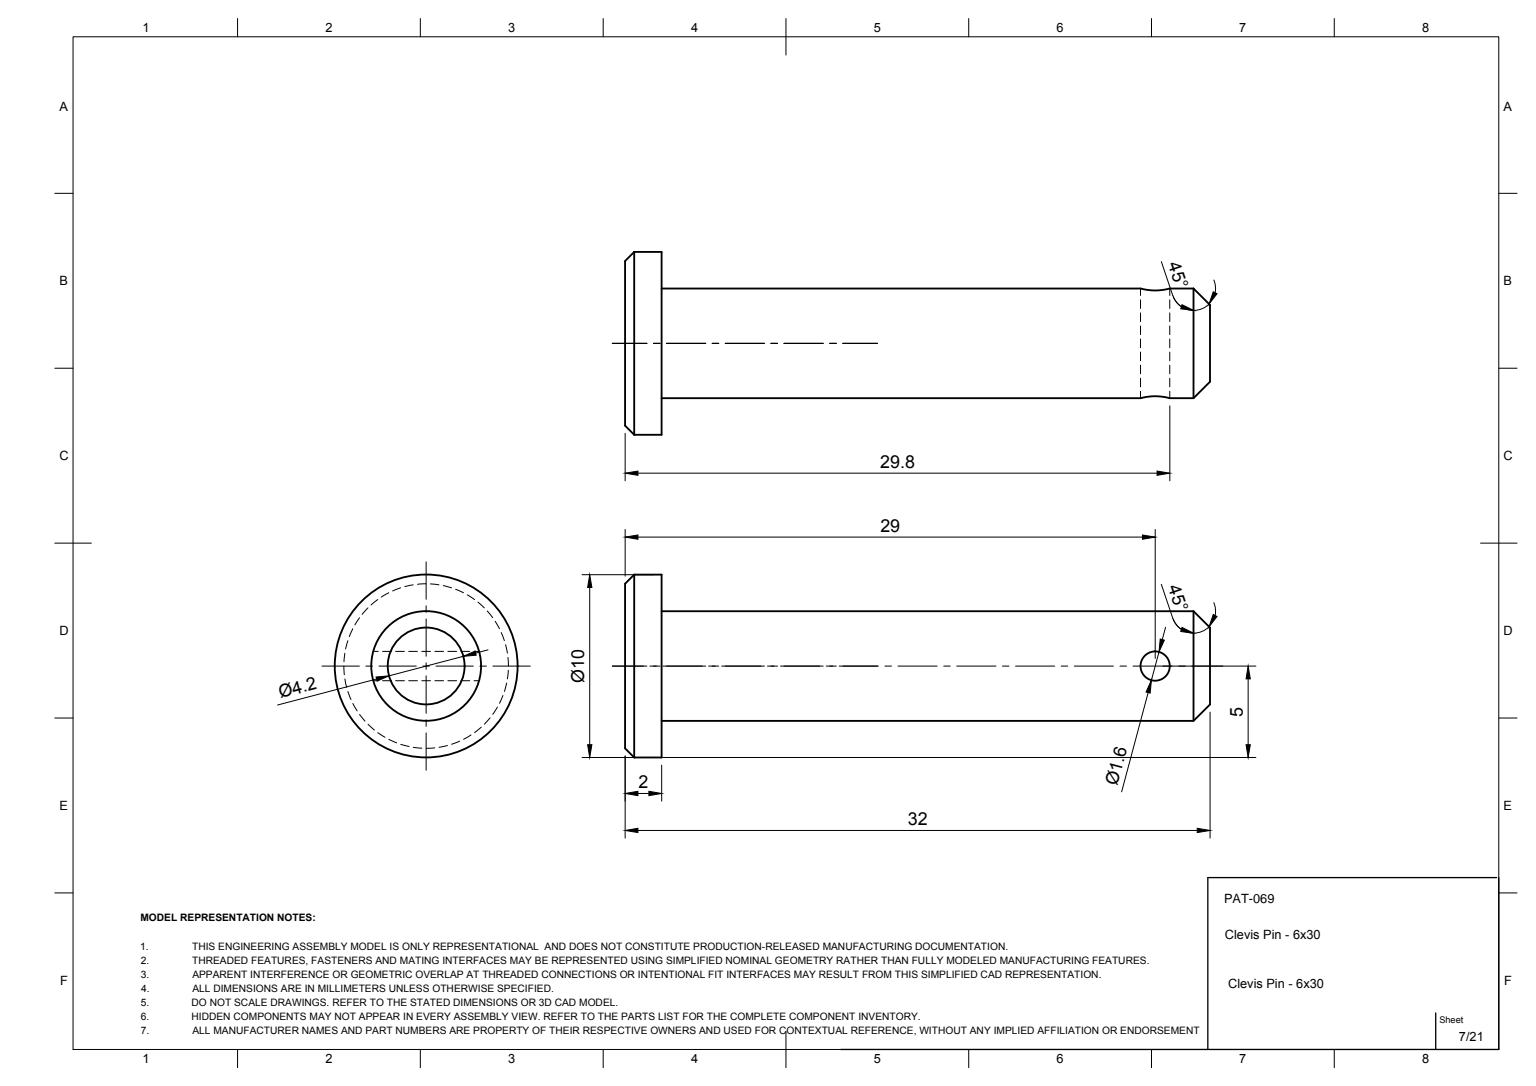
ISO-10303-21;
HEADER;
/* Generated by software containing ST-Developer
 * from STEP Tools, Inc. (www.steptools.com) 
 */

FILE_DESCRIPTION(
/* description */ ('Located fixture plate with toggle clamp'),
/* implementation_level */ '2;1');

FILE_NAME(
/* name */ 'Clevis Pin - 6x30.step',
/* time_stamp */ '2026-10-27T21:36:12-07:00',
/* author */ (''),
/* organization */ (''),
/* preprocessor_version */ 'ST-DEVELOPER v20.2',
/* originating_system */ 'Autodesk Translation Framework v15.17.0.0',
/* authorisation */ '');

FILE_SCHEMA (('AUTOMOTIVE_DESIGN { 1 0 10303 214 3 1 1 }'));
ENDSEC;

DATA;
#10=MECHANICAL_DESIGN_GEOMETRIC_PRESENTATION_REPRESENTATION('',(#341),#9285);
#12=B_SPLINE_CURVE_WITH_KNOTS('',3,(#8976,#8977,#8978,#8979,#8980,#8981,
#8982,#8983,#8984,#8985),.UNSPECIFIED.,.F.,.F.,(4,2,2,2,4),(0.,0.0302963256060356,
0.0605926512120712,0.090883446720838,0.121174242229605),.UNSPECIFIED.);
#13=B_SPLINE_CURVE_WITH_KNOTS('',3,(#8988,#8989,#8990,#8991,#8992,#8993,
#8994,#8995,#8996,#8997,#8998,#8999,#9000,#9001,#9002,#9003,#9004,#9005,
#9006,#9007,#9008,#9009,#9010,#9011,#9012,#9013,#9014,#9015,#9016,#9017,
#9018,#9019,#9020,#9021),.UNSPECIFIED.,.T.,.F.,(4,2,2,2,2,2,2,2,2,2,2,2,
2,2,2,2,4),(0.,0.0302963256060358,0.0605926512120716,0.0908834467208383,
0.121174242229605,0.151465037738372,0.181755833247138,0.212052158853174,
0.24234848445921,0.272644810065246,0.302941135671282,0.333231931180048,
0.363522726688815,0.393813522197582,0.424104317706349,0.454400643312384,
0.48469696891842),.UNSPECIFIED.);
#14=B_SPLINE_CURVE_WITH_KNOTS('',3,(#9023,#9024,#9025,#9026,#9027,#9028,
#9029,#9030,#9031,#9032),.UNSPECIFIED.,.F.,.F.,(4,2,2,2,4),(0.363522726688815,
0.393813522197581,0.424104317706348,0.454400643312384,0.48469696891842),
 .UNSPECIFIED.);
#15=B_SPLINE_CURVE_WITH_KNOTS('',3,(#9033,#9034,#9035,#9036,#9037,#9038,
#9039,#9040,#9041,#9042,#9043,#9044,#9045,#9046,#9047,#9048,#9049,#9050),
 .UNSPECIFIED.,.F.,.F.,(4,2,2,2,2,2,2,2,4),(0.121174242229605,0.151465037738371,
0.181755833247138,0.212052158853174,0.24234848445921,0.272644810065246,
0.302941135671281,0.333231931180048,0.363522726688815),.UNSPECIFIED.);
#271=CONICAL_SURFACE('',#5944,0.475,0.785398163397448);
#272=CONICAL_SURFACE('',#5952,0.255,0.785398163397449);
#293=SHAPE_REPRESENTATION_RELATIONSHIP('SRR','None',#9419,#317);
#317=ADVANCED_BREP_SHAPE_REPRESENTATION('',(#362),#9281);
#341=STYLED_ITEM('',(#9612),#362);
#362=MANIFOLD_SOLID_BREP('Body1',#5192);
#479=FACE_BOUND('',#1360,.T.);
#480=FACE_BOUND('',#1362,.T.);
#663=PLANE('',#5942);
#664=PLANE('',#5948);
#665=PLANE('',#5954);
#947=FACE_OUTER_BOUND('',#1355,.T.);
#948=FACE_OUTER_BOUND('',#1356,.T.);
#949=FACE_OUTER_BOUND('',#1357,.T.);
#950=FACE_OUTER_BOUND('',#1358,.T.);
#951=FACE_OUTER_BOUND('',#1359,.T.);
#952=FACE_OUTER_BOUND('',#1361,.T.);
#953=FACE_OUTER_BOUND('',#1363,.T.);
#954=FACE_OUTER_BOUND('',#1364,.T.);
#1355=EDGE_LOOP('',(#4712,#4713,#4714,#4715,#4716,#4717));
#1356=EDGE_LOOP('',(#4718));
#1357=EDGE_LOOP('',(#4719,#4720,#4721,#4722));
#1358=EDGE_LOOP('',(#4723,#4724,#4725,#4726));
#1359=EDGE_LOOP('',(#4727));
#1360=EDGE_LOOP('',(#4728));
#1361=EDGE_LOOP('',(#4729,#4730,#4731,#4732,#4733,#4734,#4735,#4736,#4737));
#1362=EDGE_LOOP('',(#4738));
#1363=EDGE_LOOP('',(#4739,#4740,#4741,#4742));
#1364=EDGE_LOOP('',(#4743));
#1562=CIRCLE('',#5943,0.45);
#1563=CIRCLE('',#5945,0.5);
#1564=CIRCLE('',#5947,0.5);
#1565=CIRCLE('',#5949,0.3);
#1566=CIRCLE('',#5951,0.3);
#1567=CIRCLE('',#5953,0.21);
#1976=LINE('',#8987,#2386);
#1977=LINE('',#9057,#2387);
#1978=LINE('',#9061,#2388);
#1979=LINE('',#9068,#2389);
#1980=LINE('',#9069,#2390);
#1981=LINE('',#9073,#2391);
#2386=VECTOR('',#7386,0.08);
#2387=VECTOR('',#7395,0.475);
#2388=VECTOR('',#7400,0.5);
#2389=VECTOR('',#7409,0.3);
#2390=VECTOR('',#7410,0.3);
#2391=VECTOR('',#7415,0.255);
#2804=VERTEX_POINT('',#8974);
#2805=VERTEX_POINT('',#8975);
#2806=VERTEX_POINT('',#8986);
#2807=VERTEX_POINT('',#9022);
#2808=VERTEX_POINT('',#9052);
#2809=VERTEX_POINT('',#9055);
#2810=VERTEX_POINT('',#9059);
#2811=VERTEX_POINT('',#9063);
#2812=VERTEX_POINT('',#9066);
#2813=VERTEX_POINT('',#9071);
#3444=EDGE_CURVE('',#2804,#2805,#12,.T.);
#3445=EDGE_CURVE('',#2804,#2806,#1976,.T.);
#3446=EDGE_CURVE('',#2806,#2806,#13,.T.);
#3447=EDGE_CURVE('',#2807,#2804,#14,.T.);
#3448=EDGE_CURVE('',#2805,#2807,#15,.T.);
#3449=EDGE_CURVE('',#2808,#2808,#1562,.T.);
#3450=EDGE_CURVE('',#2809,#2809,#1563,.T.);
#3451=EDGE_CURVE('',#2809,#2808,#1977,.T.);
#3452=EDGE_CURVE('',#2810,#2810,#1564,.T.);
#3453=EDGE_CURVE('',#2810,#2809,#1978,.T.);
#3454=EDGE_CURVE('',#2811,#2811,#1565,.T.);
#3455=EDGE_CURVE('',#2812,#2812,#1566,.T.);
#3456=EDGE_CURVE('',#2812,#2805,#1979,.T.);
#3457=EDGE_CURVE('',#2807,#2811,#1980,.T.);
#3458=EDGE_CURVE('',#2813,#2813,#1567,.T.);
#3459=EDGE_CURVE('',#2813,#2812,#1981,.T.);
#4712=ORIENTED_EDGE('',*,*,#3444,.F.);
#4713=ORIENTED_EDGE('',*,*,#3445,.T.);
#4714=ORIENTED_EDGE('',*,*,#3446,.F.);
#4715=ORIENTED_EDGE('',*,*,#3445,.F.);
#4716=ORIENTED_EDGE('',*,*,#3447,.F.);
#4717=ORIENTED_EDGE('',*,*,#3448,.F.);
#4718=ORIENTED_EDGE('',*,*,#3449,.F.);
#4719=ORIENTED_EDGE('',*,*,#3450,.F.);
#4720=ORIENTED_EDGE('',*,*,#3451,.T.);
#4721=ORIENTED_EDGE('',*,*,#3449,.T.);
#4722=ORIENTED_EDGE('',*,*,#3451,.F.);
#4723=ORIENTED_EDGE('',*,*,#3452,.F.);
#4724=ORIENTED_EDGE('',*,*,#3453,.T.);
#4725=ORIENTED_EDGE('',*,*,#3450,.T.);
#4726=ORIENTED_EDGE('',*,*,#3453,.F.);
#4727=ORIENTED_EDGE('',*,*,#3452,.T.);
#4728=ORIENTED_EDGE('',*,*,#3454,.F.);
#4729=ORIENTED_EDGE('',*,*,#3455,.F.);
#4730=ORIENTED_EDGE('',*,*,#3456,.T.);
#4731=ORIENTED_EDGE('',*,*,#3448,.T.);
#4732=ORIENTED_EDGE('',*,*,#3457,.T.);
#4733=ORIENTED_EDGE('',*,*,#3454,.T.);
#4734=ORIENTED_EDGE('',*,*,#3457,.F.);
#4735=ORIENTED_EDGE('',*,*,#3447,.T.);
#4736=ORIENTED_EDGE('',*,*,#3444,.T.);
#4737=ORIENTED_EDGE('',*,*,#3456,.F.);
#4738=ORIENTED_EDGE('',*,*,#3446,.T.);
#4739=ORIENTED_EDGE('',*,*,#3458,.F.);
#4740=ORIENTED_EDGE('',*,*,#3459,.T.);
#4741=ORIENTED_EDGE('',*,*,#3455,.T.);
#4742=ORIENTED_EDGE('',*,*,#3459,.F.);
#4743=ORIENTED_EDGE('',*,*,#3458,.T.);
#4866=CYLINDRICAL_SURFACE('',#5941,0.08);
#4867=CYLINDRICAL_SURFACE('',#5946,0.5);
#4868=CYLINDRICAL_SURFACE('',#5950,0.3);
#5148=ADVANCED_FACE('',(#947),#4866,.F.);
#5149=ADVANCED_FACE('',(#948),#663,.T.);
#5150=ADVANCED_FACE('',(#949),#271,.T.);
#5151=ADVANCED_FACE('',(#950),#4867,.T.);
#5152=ADVANCED_FACE('',(#951,#479),#664,.T.);
#5153=ADVANCED_FACE('',(#952,#480),#4868,.T.);
#5154=ADVANCED_FACE('',(#953),#272,.T.);
#5155=ADVANCED_FACE('',(#954),#665,.T.);
#5192=CLOSED_SHELL('',(#5148,#5149,#5150,#5151,#5152,#5153,#5154,#5155));
#5940=AXIS2_PLACEMENT_3D('',#8972,#7382,#7383);
#5941=AXIS2_PLACEMENT_3D('',#8973,#7384,#7385);
#5942=AXIS2_PLACEMENT_3D('',#9051,#7387,#7388);
#5943=AXIS2_PLACEMENT_3D('',#9053,#7389,#7390);
#5944=AXIS2_PLACEMENT_3D('',#9054,#7391,#7392);
#5945=AXIS2_PLACEMENT_3D('',#9056,#7393,#7394);
#5946=AXIS2_PLACEMENT_3D('',#9058,#7396,#7397);
#5947=AXIS2_PLACEMENT_3D('',#9060,#7398,#7399);
#5948=AXIS2_PLACEMENT_3D('',#9062,#7401,#7402);
#5949=AXIS2_PLACEMENT_3D('',#9064,#7403,#7404);
#5950=AXIS2_PLACEMENT_3D('',#9065,#7405,#7406);
#5951=AXIS2_PLACEMENT_3D('',#9067,#7407,#7408);
#5952=AXIS2_PLACEMENT_3D('',#9070,#7411,#7412);
#5953=AXIS2_PLACEMENT_3D('',#9072,#7413,#7414);
#5954=AXIS2_PLACEMENT_3D('',#9074,#7416,#7417);
#7382=DIRECTION('axis',(0.,0.,1.));
#7383=DIRECTION('refdir',(1.,0.,0.));
#7384=DIRECTION('center_axis',(1.,0.,0.));
#7385=DIRECTION('ref_axis',(0.,0.,-1.));
#7386=DIRECTION('',(1.,0.,0.));
#7387=DIRECTION('center_axis',(0.,1.,0.));
#7388=DIRECTION('ref_axis',(0.,0.,1.));
#7389=DIRECTION('center_axis',(0.,-1.,0.));
#7390=DIRECTION('ref_axis',(1.,0.,0.));
#7391=DIRECTION('center_axis',(0.,-1.,0.));
#7392=DIRECTION('ref_axis',(1.,0.,0.));
#7393=DIRECTION('center_axis',(0.,-1.,0.));
#7394=DIRECTION('ref_axis',(1.,0.,0.));
#7395=DIRECTION('',(0.707106781186547,0.707106781186548,8.65956056235493E-17));
#7396=DIRECTION('center_axis',(0.,-1.,0.));
#7397=DIRECTION('ref_axis',(1.,0.,0.));
#7398=DIRECTION('center_axis',(0.,-1.,0.));
#7399=DIRECTION('ref_axis',(1.,0.,0.));
#7400=DIRECTION('',(0.,1.,0.));
#7401=DIRECTION('center_axis',(0.,-1.,0.));
#7402=DIRECTION('ref_axis',(0.,0.,-1.));
#7403=DIRECTION('center_axis',(0.,-1.,0.));
#7404=DIRECTION('ref_axis',(1.,0.,0.));
#7405=DIRECTION('center_axis',(0.,-1.,0.));
#7406=DIRECTION('ref_axis',(1.,0.,0.));
#7407=DIRECTION('center_axis',(0.,-1.,0.));
#7408=DIRECTION('ref_axis',(1.,0.,0.));
#7409=DIRECTION('',(0.,1.,0.));
#7410=DIRECTION('',(0.,1.,0.));
#7411=DIRECTION('center_axis',(0.,1.,0.));
#7412=DIRECTION('ref_axis',(1.,0.,0.));
#7413=DIRECTION('center_axis',(0.,-1.,0.));
#7414=DIRECTION('ref_axis',(1.,0.,0.));
#7415=DIRECTION('',(-0.707106781186548,0.707106781186547,-8.65956056235494E-17));
#7416=DIRECTION('center_axis',(0.,-1.,0.));
#7417=DIRECTION('ref_axis',(0.,0.,-1.));
#8972=CARTESIAN_POINT('',(0.,0.,0.));
#8973=CARTESIAN_POINT('Origin',(0.,-2.7,0.));
#8974=CARTESIAN_POINT('',(-0.289136645896019,-2.7,0.08));
#8975=CARTESIAN_POINT('',(-0.3,-2.78,-2.27065106771523E-17));
#8976=CARTESIAN_POINT('Ctrl Pts',(-0.289136645896019,-2.7,0.08));
#8977=CARTESIAN_POINT('Ctrl Pts',(-0.289136645896019,-2.71009877520201,
0.08));
#8978=CARTESIAN_POINT('Ctrl Pts',(-0.289720927595908,-2.72083518625944,
0.0779717130936404));
#8979=CARTESIAN_POINT('Ctrl Pts',(-0.291799203044223,-2.74052980652726,
0.0697927537456149));
#8980=CARTESIAN_POINT('Ctrl Pts',(-0.293259762986909,-2.74949254880105,
0.0636445361887959));
#8981=CARTESIAN_POINT('Ctrl Pts',(-0.295976783522942,-2.76364324458222,
0.0494938404076284));
#8982=CARTESIAN_POINT('Ctrl Pts',(-0.297414335384467,-2.76979246713824,
0.0405305642602551));
#8983=CARTESIAN_POINT('Ctrl Pts',(-0.299439403644655,-2.77797216257078,
0.0208340363410407));
#8984=CARTESIAN_POINT('Ctrl Pts',(-0.3,-2.78,0.0100969318362556));
#8985=CARTESIAN_POINT('Ctrl Pts',(-0.3,-2.78,5.20417042793042E-18));
#8986=CARTESIAN_POINT('',(0.289136645896019,-2.7,0.08));
#8987=CARTESIAN_POINT('',(0.,-2.7,0.08));
#8988=CARTESIAN_POINT('Ctrl Pts',(0.289136645896019,-2.7,0.08));
#8989=CARTESIAN_POINT('Ctrl Pts',(0.289136645896019,-2.68990122479799,0.08));
#8990=CARTESIAN_POINT('Ctrl Pts',(0.289720927595908,-2.67916481374056,0.0779717130936404));
#8991=CARTESIAN_POINT('Ctrl Pts',(0.291799203044223,-2.65947019347274,0.0697927537456147));
#8992=CARTESIAN_POINT('Ctrl Pts',(0.293259762986909,-2.65050745119895,0.0636445361887959));
#8993=CARTESIAN_POINT('Ctrl Pts',(0.295976783522942,-2.63635675541778,0.0494938404076283));
#8994=CARTESIAN_POINT('Ctrl Pts',(0.297414335384467,-2.63020753286176,0.0405305642602551));
#8995=CARTESIAN_POINT('Ctrl Pts',(0.299439403644655,-2.62202783742922,0.0208340363410406));
#8996=CARTESIAN_POINT('Ctrl Pts',(0.3,-2.62,0.0100969318362555));
#8997=CARTESIAN_POINT('Ctrl Pts',(0.3,-2.62,-0.0100969318362556));
#8998=CARTESIAN_POINT('Ctrl Pts',(0.299439403644655,-2.62202783742922,-0.0208340363410406));
#8999=CARTESIAN_POINT('Ctrl Pts',(0.297414335384467,-2.63020753286176,-0.0405305642602551));
#9000=CARTESIAN_POINT('Ctrl Pts',(0.295976783522942,-2.63635675541778,-0.0494938404076283));
#9001=CARTESIAN_POINT('Ctrl Pts',(0.293259762986909,-2.65050745119895,-0.0636445361887959));
#9002=CARTESIAN_POINT('Ctrl Pts',(0.291799203044223,-2.65947019347274,-0.0697927537456147));
#9003=CARTESIAN_POINT('Ctrl Pts',(0.289720927595908,-2.67916481374056,-0.0779717130936403));
#9004=CARTESIAN_POINT('Ctrl Pts',(0.289136645896019,-2.68990122479799,-0.08));
#9005=CARTESIAN_POINT('Ctrl Pts',(0.289136645896019,-2.71009877520201,-0.08));
#9006=CARTESIAN_POINT('Ctrl Pts',(0.289720927595908,-2.72083518625944,-0.0779717130936404));
#9007=CARTESIAN_POINT('Ctrl Pts',(0.291799203044223,-2.74052980652726,-0.0697927537456147));
#9008=CARTESIAN_POINT('Ctrl Pts',(0.293259762986909,-2.74949254880105,-0.0636445361887959));
#9009=CARTESIAN_POINT('Ctrl Pts',(0.295976783522942,-2.76364324458222,-0.0494938404076283));
#9010=CARTESIAN_POINT('Ctrl Pts',(0.297414335384467,-2.76979246713824,-0.0405305642602551));
#9011=CARTESIAN_POINT('Ctrl Pts',(0.299439403644655,-2.77797216257078,-0.0208340363410406));
#9012=CARTESIAN_POINT('Ctrl Pts',(0.3,-2.78,-0.0100969318362555));
#9013=CARTESIAN_POINT('Ctrl Pts',(0.3,-2.78,0.0100969318362556));
#9014=CARTESIAN_POINT('Ctrl Pts',(0.299439403644655,-2.77797216257078,0.0208340363410407));
#9015=CARTESIAN_POINT('Ctrl Pts',(0.297414335384467,-2.76979246713824,0.0405305642602551));
#9016=CARTESIAN_POINT('Ctrl Pts',(0.295976783522942,-2.76364324458222,0.0494938404076284));
#9017=CARTESIAN_POINT('Ctrl Pts',(0.293259762986909,-2.74949254880105,0.0636445361887959));
#9018=CARTESIAN_POINT('Ctrl Pts',(0.291799203044223,-2.74052980652726,0.0697927537456149));
#9019=CARTESIAN_POINT('Ctrl Pts',(0.289720927595908,-2.72083518625944,0.0779717130936404));
#9020=CARTESIAN_POINT('Ctrl Pts',(0.289136645896019,-2.71009877520201,0.08));
#9021=CARTESIAN_POINT('Ctrl Pts',(0.289136645896019,-2.7,0.08));
#9022=CARTESIAN_POINT('',(-0.3,-2.62,-3.65842984849668E-17));
#9023=CARTESIAN_POINT('Ctrl Pts',(-0.3,-2.62,-3.81639164714898E-17));
#9024=CARTESIAN_POINT('Ctrl Pts',(-0.3,-2.62,0.0100969318362555));
#9025=CARTESIAN_POINT('Ctrl Pts',(-0.299439403644655,-2.62202783742922,
0.0208340363410406));
#9026=CARTESIAN_POINT('Ctrl Pts',(-0.297414335384467,-2.63020753286176,
0.040530564260255));
#9027=CARTESIAN_POINT('Ctrl Pts',(-0.295976783522942,-2.63635675541778,
0.0494938404076283));
#9028=CARTESIAN_POINT('Ctrl Pts',(-0.293259762986909,-2.65050745119895,
0.0636445361887959));
#9029=CARTESIAN_POINT('Ctrl Pts',(-0.291799203044223,-2.65947019347274,
0.0697927537456147));
#9030=CARTESIAN_POINT('Ctrl Pts',(-0.289720927595908,-2.67916481374056,
0.0779717130936404));
#9031=CARTESIAN_POINT('Ctrl Pts',(-0.289136645896019,-2.68990122479799,
0.08));
#9032=CARTESIAN_POINT('Ctrl Pts',(-0.289136645896019,-2.7,0.08));
#9033=CARTESIAN_POINT('Ctrl Pts',(-0.3,-2.78,-6.93889390390723E-18));
#9034=CARTESIAN_POINT('Ctrl Pts',(-0.3,-2.78,-0.0100969318362556));
#9035=CARTESIAN_POINT('Ctrl Pts',(-0.299439403644655,-2.77797216257078,
-0.0208340363410406));
#9036=CARTESIAN_POINT('Ctrl Pts',(-0.297414335384467,-2.76979246713824,
-0.0405305642602551));
#9037=CARTESIAN_POINT('Ctrl Pts',(-0.295976783522942,-2.76364324458222,
-0.0494938404076283));
#9038=CARTESIAN_POINT('Ctrl Pts',(-0.293259762986909,-2.74949254880105,
-0.0636445361887959));
#9039=CARTESIAN_POINT('Ctrl Pts',(-0.291799203044223,-2.74052980652726,
-0.0697927537456147));
#9040=CARTESIAN_POINT('Ctrl Pts',(-0.289720927595908,-2.72083518625944,
-0.0779717130936403));
#9041=CARTESIAN_POINT('Ctrl Pts',(-0.289136645896019,-2.71009877520201,
-0.08));
#9042=CARTESIAN_POINT('Ctrl Pts',(-0.289136645896019,-2.68990122479799,
-0.08));
#9043=CARTESIAN_POINT('Ctrl Pts',(-0.289720927595908,-2.67916481374056,
-0.0779717130936403));
#9044=CARTESIAN_POINT('Ctrl Pts',(-0.291799203044223,-2.65947019347274,
-0.0697927537456147));
#9045=CARTESIAN_POINT('Ctrl Pts',(-0.293259762986909,-2.65050745119895,
-0.0636445361887959));
#9046=CARTESIAN_POINT('Ctrl Pts',(-0.295976783522942,-2.63635675541778,
-0.0494938404076283));
#9047=CARTESIAN_POINT('Ctrl Pts',(-0.297414335384467,-2.63020753286176,
-0.0405305642602551));
#9048=CARTESIAN_POINT('Ctrl Pts',(-0.299439403644655,-2.62202783742922,
-0.0208340363410406));
#9049=CARTESIAN_POINT('Ctrl Pts',(-0.3,-2.62,-0.0100969318362556));
#9050=CARTESIAN_POINT('Ctrl Pts',(-0.3,-2.62,-1.56125112837913E-17));
#9051=CARTESIAN_POINT('Origin',(0.45,0.2,0.));
#9052=CARTESIAN_POINT('',(-0.45,0.2,-5.51091059616309E-17));
#9053=CARTESIAN_POINT('Origin',(0.,0.2,0.));
#9054=CARTESIAN_POINT('Origin',(0.,0.175,0.));
#9055=CARTESIAN_POINT('',(-0.5,0.15,-6.12323399573676E-17));
#9056=CARTESIAN_POINT('Origin',(0.,0.15,0.));
#9057=CARTESIAN_POINT('',(-0.475,0.175,-5.81707229594993E-17));
#9058=CARTESIAN_POINT('Origin',(0.,0.0750000000000002,0.));
#9059=CARTESIAN_POINT('',(-0.5,0.,-6.12323399573677E-17));
#9060=CARTESIAN_POINT('Origin',(0.,0.,0.));
#9061=CARTESIAN_POINT('',(-0.5,0.0750000000000002,-6.12323399573677E-17));
#9062=CARTESIAN_POINT('Origin',(0.3,0.,0.));
#9063=CARTESIAN_POINT('',(-0.3,0.,-3.67394039744206E-17));
#9064=CARTESIAN_POINT('Origin',(0.,0.,0.));
#9065=CARTESIAN_POINT('Origin',(0.,-1.455,0.));
#9066=CARTESIAN_POINT('',(-0.3,-2.91,-3.67394039744206E-17));
#9067=CARTESIAN_POINT('Origin',(0.,-2.91,0.));
#9068=CARTESIAN_POINT('',(-0.3,-1.455,-3.67394039744206E-17));
#9069=CARTESIAN_POINT('',(-0.3,-1.455,-3.67394039744206E-17));
#9070=CARTESIAN_POINT('Origin',(0.,-2.955,0.));
#9071=CARTESIAN_POINT('',(-0.21,-3.,-2.57175827820944E-17));
#9072=CARTESIAN_POINT('Origin',(0.,-3.,0.));
#9073=CARTESIAN_POINT('',(-0.255,-2.955,-3.12284933782575E-17));
#9074=CARTESIAN_POINT('Origin',(0.,-3.,0.));
#9251=UNCERTAINTY_MEASURE_WITH_UNIT(LENGTH_MEASURE(0.001),#9286,
'DISTANCE_ACCURACY_VALUE',
'Maximum model space distance between geometric entities at asserted c
onnectivities');
#9255=UNCERTAINTY_MEASURE_WITH_UNIT(LENGTH_MEASURE(0.001),#9286,
'DISTANCE_ACCURACY_VALUE',
'Maximum model space distance between geometric entities at asserted c
onnectivities');
#9281=(
GEOMETRIC_REPRESENTATION_CONTEXT(3)
GLOBAL_UNCERTAINTY_ASSIGNED_CONTEXT((#9251))
GLOBAL_UNIT_ASSIGNED_CONTEXT((#9286,#9288,#9289))
REPRESENTATION_CONTEXT('','3D')
);
#9285=(
GEOMETRIC_REPRESENTATION_CONTEXT(3)
GLOBAL_UNCERTAINTY_ASSIGNED_CONTEXT((#9255))
GLOBAL_UNIT_ASSIGNED_CONTEXT((#9286,#9288,#9289))
REPRESENTATION_CONTEXT('','3D')
);
#9286=(
LENGTH_UNIT()
NAMED_UNIT(*)
SI_UNIT(.CENTI.,.METRE.)
);
#9288=(
NAMED_UNIT(*)
PLANE_ANGLE_UNIT()
SI_UNIT($,.RADIAN.)
);
#9289=(
NAMED_UNIT(*)
SI_UNIT($,.STERADIAN.)
SOLID_ANGLE_UNIT()
);
#9315=SHAPE_DEFINITION_REPRESENTATION(#9345,#9419);
#9345=PRODUCT_DEFINITION_SHAPE('',$,#9449);
#9419=SHAPE_REPRESENTATION('',(#5940),#9281);
#9423=PRODUCT_DEFINITION_CONTEXT('part definition',#9512,'design');
#9449=PRODUCT_DEFINITION('Clevis Pin - 6x30','Clevis Pin - 6x30',#9478,
#9423);
#9478=PRODUCT_DEFINITION_FORMATION('',$,#9539);
#9512=APPLICATION_CONTEXT(
'Core Data for Automotive Mechanical Design Process');
#9513=PRODUCT_CONTEXT('part definition',#9512,'mechanical');
#9539=PRODUCT('Clevis Pin - 6x30','Clevis Pin - 6x30',
'Clevis Pin - 6x30',(#9513));
#9606=COLOUR_RGB('Grey',0.48,0.52,0.57);
#9607=FILL_AREA_STYLE_COLOUR('',#9606);
#9608=FILL_AREA_STYLE('',(#9607));
#9609=SURFACE_STYLE_FILL_AREA(#9608);
#9610=SURFACE_SIDE_STYLE('',(#9609));
#9611=SURFACE_STYLE_USAGE(.BOTH.,#9610);
#9612=PRESENTATION_STYLE_ASSIGNMENT((#9611));
ENDSEC;
END-ISO-10303-21;
